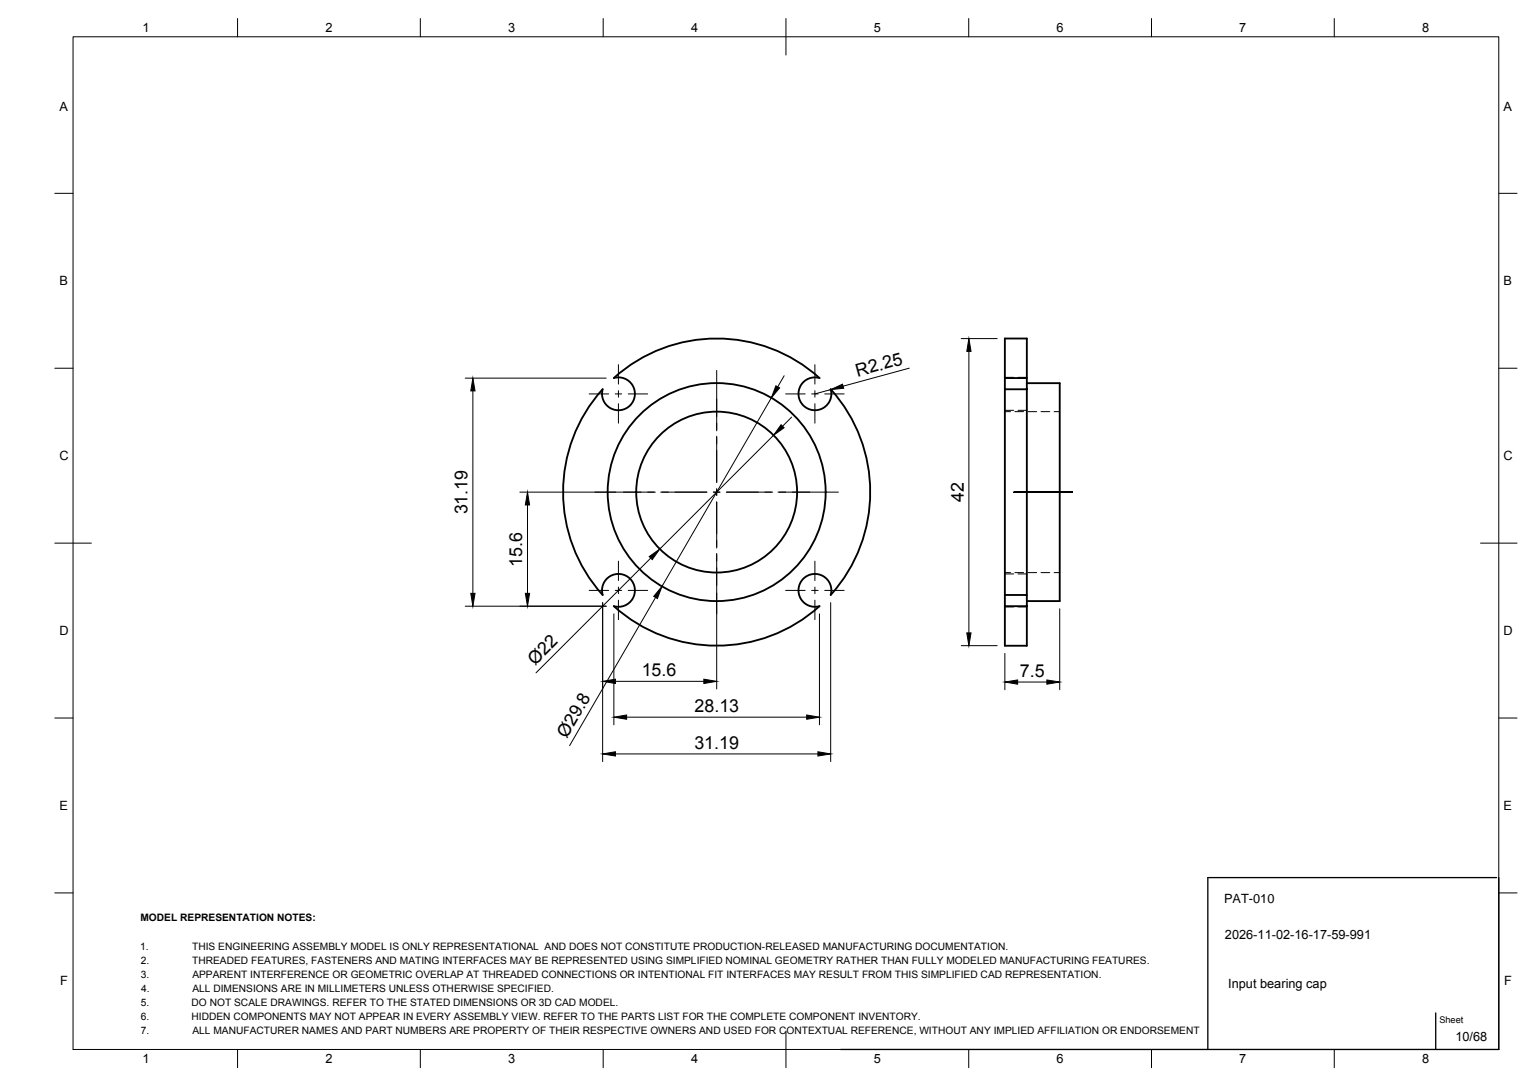
ISO-10303-21;
HEADER;
/* Generated by software containing ST-Developer
 * from STEP Tools, Inc. (www.steptools.com) 
 */

FILE_DESCRIPTION(
/* description */ ('Belt conveyor head drive unit'),
/* implementation_level */ '2;1');

FILE_NAME(
/* name */ 'Input bearing cap.step',
/* time_stamp */ '2026-10-28T03:26:19-07:00',
/* author */ (''),
/* organization */ (''),
/* preprocessor_version */ 'ST-DEVELOPER v20.2',
/* originating_system */ 'Autodesk Translation Framework v15.17.0.0',
/* authorisation */ '');

FILE_SCHEMA (('AUTOMOTIVE_DESIGN { 1 0 10303 214 3 1 1 }'));
ENDSEC;

DATA;
#10=MECHANICAL_DESIGN_GEOMETRIC_PRESENTATION_REPRESENTATION('',(#852),#27069);
#714=SHAPE_REPRESENTATION_RELATIONSHIP('SRR','None',#27358,#783);
#783=ADVANCED_BREP_SHAPE_REPRESENTATION('',(#937),#27000);
#852=STYLED_ITEM('',(#27797),#937);
#937=MANIFOLD_SOLID_BREP('Body1',#13717);
#1052=FACE_BOUND('',#2563,.T.);
#1053=FACE_BOUND('',#2570,.T.);
#1054=FACE_BOUND('',#2573,.T.);
#1329=PLANE('',#14737);
#1330=PLANE('',#14754);
#1331=PLANE('',#14757);
#1718=FACE_OUTER_BOUND('',#2558,.T.);
#1719=FACE_OUTER_BOUND('',#2559,.T.);
#1720=FACE_OUTER_BOUND('',#2560,.T.);
#1721=FACE_OUTER_BOUND('',#2561,.T.);
#1722=FACE_OUTER_BOUND('',#2562,.T.);
#1723=FACE_OUTER_BOUND('',#2564,.T.);
#1724=FACE_OUTER_BOUND('',#2565,.T.);
#1725=FACE_OUTER_BOUND('',#2566,.T.);
#1726=FACE_OUTER_BOUND('',#2567,.T.);
#1727=FACE_OUTER_BOUND('',#2568,.T.);
#1728=FACE_OUTER_BOUND('',#2569,.T.);
#1729=FACE_OUTER_BOUND('',#2571,.T.);
#1730=FACE_OUTER_BOUND('',#2572,.T.);
#2558=EDGE_LOOP('',(#9336,#9337,#9338,#9339));
#2559=EDGE_LOOP('',(#9340,#9341,#9342,#9343));
#2560=EDGE_LOOP('',(#9344,#9345,#9346,#9347));
#2561=EDGE_LOOP('',(#9348,#9349,#9350,#9351));
#2562=EDGE_LOOP('',(#9352,#9353,#9354,#9355,#9356,#9357,#9358,#9359));
#2563=EDGE_LOOP('',(#9360));
#2564=EDGE_LOOP('',(#9361,#9362,#9363,#9364));
#2565=EDGE_LOOP('',(#9365,#9366,#9367,#9368));
#2566=EDGE_LOOP('',(#9369,#9370,#9371,#9372));
#2567=EDGE_LOOP('',(#9373,#9374,#9375,#9376));
#2568=EDGE_LOOP('',(#9377,#9378,#9379,#9380));
#2569=EDGE_LOOP('',(#9381));
#2570=EDGE_LOOP('',(#9382));
#2571=EDGE_LOOP('',(#9383,#9384,#9385,#9386));
#2572=EDGE_LOOP('',(#9387,#9388,#9389,#9390,#9391,#9392,#9393,#9394));
#2573=EDGE_LOOP('',(#9395));
#3617=LINE('',#21381,#4409);
#3618=LINE('',#21385,#4410);
#3619=LINE('',#21390,#4411);
#3620=LINE('',#21394,#4412);
#3621=LINE('',#21399,#4413);
#3622=LINE('',#21403,#4414);
#3623=LINE('',#21408,#4415);
#3624=LINE('',#21412,#4416);
#3625=LINE('',#21433,#4417);
#3626=LINE('',#21439,#4418);
#4409=VECTOR('',#16881,1.);
#4410=VECTOR('',#16884,1.);
#4411=VECTOR('',#16889,1.);
#4412=VECTOR('',#16892,1.);
#4413=VECTOR('',#16897,1.);
#4414=VECTOR('',#16900,1.);
#4415=VECTOR('',#16905,1.);
#4416=VECTOR('',#16908,1.);
#4417=VECTOR('',#16943,1.49);
#4418=VECTOR('',#16952,1.1);
#5152=CIRCLE('',#14726,0.225);
#5153=CIRCLE('',#14727,0.225);
#5154=CIRCLE('',#14729,0.225);
#5155=CIRCLE('',#14730,0.225);
#5156=CIRCLE('',#14732,0.225);
#5157=CIRCLE('',#14733,0.225);
#5158=CIRCLE('',#14735,0.225);
#5159=CIRCLE('',#14736,0.225);
#5160=CIRCLE('',#14738,2.1);
#5161=CIRCLE('',#14739,2.1);
#5162=CIRCLE('',#14740,2.1);
#5163=CIRCLE('',#14741,2.1);
#5164=CIRCLE('',#14742,1.1);
#5165=CIRCLE('',#14744,2.1);
#5166=CIRCLE('',#14746,2.1);
#5167=CIRCLE('',#14748,2.1);
#5168=CIRCLE('',#14750,2.1);
#5169=CIRCLE('',#14752,1.49);
#5170=CIRCLE('',#14753,1.49);
#5171=CIRCLE('',#14755,1.1);
#6079=VERTEX_POINT('',#21379);
#6080=VERTEX_POINT('',#21380);
#6081=VERTEX_POINT('',#21382);
#6082=VERTEX_POINT('',#21384);
#6083=VERTEX_POINT('',#21388);
#6084=VERTEX_POINT('',#21389);
#6085=VERTEX_POINT('',#21391);
#6086=VERTEX_POINT('',#21393);
#6087=VERTEX_POINT('',#21397);
#6088=VERTEX_POINT('',#21398);
#6089=VERTEX_POINT('',#21400);
#6090=VERTEX_POINT('',#21402);
#6091=VERTEX_POINT('',#21406);
#6092=VERTEX_POINT('',#21407);
#6093=VERTEX_POINT('',#21409);
#6094=VERTEX_POINT('',#21411);
#6095=VERTEX_POINT('',#21419);
#6096=VERTEX_POINT('',#21430);
#6097=VERTEX_POINT('',#21432);
#6098=VERTEX_POINT('',#21436);
#7360=EDGE_CURVE('',#6079,#6080,#3617,.T.);
#7361=EDGE_CURVE('',#6081,#6079,#5152,.T.);
#7362=EDGE_CURVE('',#6082,#6081,#3618,.T.);
#7363=EDGE_CURVE('',#6080,#6082,#5153,.T.);
#7364=EDGE_CURVE('',#6083,#6084,#3619,.T.);
#7365=EDGE_CURVE('',#6085,#6083,#5154,.T.);
#7366=EDGE_CURVE('',#6086,#6085,#3620,.T.);
#7367=EDGE_CURVE('',#6084,#6086,#5155,.T.);
#7368=EDGE_CURVE('',#6087,#6088,#3621,.T.);
#7369=EDGE_CURVE('',#6089,#6087,#5156,.T.);
#7370=EDGE_CURVE('',#6090,#6089,#3622,.T.);
#7371=EDGE_CURVE('',#6088,#6090,#5157,.T.);
#7372=EDGE_CURVE('',#6091,#6092,#3623,.T.);
#7373=EDGE_CURVE('',#6093,#6091,#5158,.T.);
#7374=EDGE_CURVE('',#6094,#6093,#3624,.T.);
#7375=EDGE_CURVE('',#6092,#6094,#5159,.T.);
#7376=EDGE_CURVE('',#6093,#6079,#5160,.T.);
#7377=EDGE_CURVE('',#6089,#6091,#5161,.T.);
#7378=EDGE_CURVE('',#6085,#6087,#5162,.T.);
#7379=EDGE_CURVE('',#6081,#6083,#5163,.T.);
#7380=EDGE_CURVE('',#6095,#6095,#5164,.T.);
#7381=EDGE_CURVE('',#6090,#6092,#5165,.T.);
#7382=EDGE_CURVE('',#6086,#6088,#5166,.T.);
#7383=EDGE_CURVE('',#6094,#6080,#5167,.T.);
#7384=EDGE_CURVE('',#6082,#6084,#5168,.T.);
#7385=EDGE_CURVE('',#6096,#6096,#5169,.T.);
#7386=EDGE_CURVE('',#6096,#6097,#3625,.T.);
#7387=EDGE_CURVE('',#6097,#6097,#5170,.T.);
#7388=EDGE_CURVE('',#6098,#6098,#5171,.T.);
#7389=EDGE_CURVE('',#6098,#6095,#3626,.T.);
#9336=ORIENTED_EDGE('',*,*,#7360,.F.);
#9337=ORIENTED_EDGE('',*,*,#7361,.F.);
#9338=ORIENTED_EDGE('',*,*,#7362,.F.);
#9339=ORIENTED_EDGE('',*,*,#7363,.F.);
#9340=ORIENTED_EDGE('',*,*,#7364,.F.);
#9341=ORIENTED_EDGE('',*,*,#7365,.F.);
#9342=ORIENTED_EDGE('',*,*,#7366,.F.);
#9343=ORIENTED_EDGE('',*,*,#7367,.F.);
#9344=ORIENTED_EDGE('',*,*,#7368,.F.);
#9345=ORIENTED_EDGE('',*,*,#7369,.F.);
#9346=ORIENTED_EDGE('',*,*,#7370,.F.);
#9347=ORIENTED_EDGE('',*,*,#7371,.F.);
#9348=ORIENTED_EDGE('',*,*,#7372,.F.);
#9349=ORIENTED_EDGE('',*,*,#7373,.F.);
#9350=ORIENTED_EDGE('',*,*,#7374,.F.);
#9351=ORIENTED_EDGE('',*,*,#7375,.F.);
#9352=ORIENTED_EDGE('',*,*,#7361,.T.);
#9353=ORIENTED_EDGE('',*,*,#7376,.F.);
#9354=ORIENTED_EDGE('',*,*,#7373,.T.);
#9355=ORIENTED_EDGE('',*,*,#7377,.F.);
#9356=ORIENTED_EDGE('',*,*,#7369,.T.);
#9357=ORIENTED_EDGE('',*,*,#7378,.F.);
#9358=ORIENTED_EDGE('',*,*,#7365,.T.);
#9359=ORIENTED_EDGE('',*,*,#7379,.F.);
#9360=ORIENTED_EDGE('',*,*,#7380,.F.);
#9361=ORIENTED_EDGE('',*,*,#7370,.T.);
#9362=ORIENTED_EDGE('',*,*,#7377,.T.);
#9363=ORIENTED_EDGE('',*,*,#7372,.T.);
#9364=ORIENTED_EDGE('',*,*,#7381,.F.);
#9365=ORIENTED_EDGE('',*,*,#7366,.T.);
#9366=ORIENTED_EDGE('',*,*,#7378,.T.);
#9367=ORIENTED_EDGE('',*,*,#7368,.T.);
#9368=ORIENTED_EDGE('',*,*,#7382,.F.);
#9369=ORIENTED_EDGE('',*,*,#7360,.T.);
#9370=ORIENTED_EDGE('',*,*,#7383,.F.);
#9371=ORIENTED_EDGE('',*,*,#7374,.T.);
#9372=ORIENTED_EDGE('',*,*,#7376,.T.);
#9373=ORIENTED_EDGE('',*,*,#7362,.T.);
#9374=ORIENTED_EDGE('',*,*,#7379,.T.);
#9375=ORIENTED_EDGE('',*,*,#7364,.T.);
#9376=ORIENTED_EDGE('',*,*,#7384,.F.);
#9377=ORIENTED_EDGE('',*,*,#7385,.F.);
#9378=ORIENTED_EDGE('',*,*,#7386,.T.);
#9379=ORIENTED_EDGE('',*,*,#7387,.F.);
#9380=ORIENTED_EDGE('',*,*,#7386,.F.);
#9381=ORIENTED_EDGE('',*,*,#7385,.T.);
#9382=ORIENTED_EDGE('',*,*,#7388,.T.);
#9383=ORIENTED_EDGE('',*,*,#7388,.F.);
#9384=ORIENTED_EDGE('',*,*,#7389,.T.);
#9385=ORIENTED_EDGE('',*,*,#7380,.T.);
#9386=ORIENTED_EDGE('',*,*,#7389,.F.);
#9387=ORIENTED_EDGE('',*,*,#7363,.T.);
#9388=ORIENTED_EDGE('',*,*,#7384,.T.);
#9389=ORIENTED_EDGE('',*,*,#7367,.T.);
#9390=ORIENTED_EDGE('',*,*,#7382,.T.);
#9391=ORIENTED_EDGE('',*,*,#7371,.T.);
#9392=ORIENTED_EDGE('',*,*,#7381,.T.);
#9393=ORIENTED_EDGE('',*,*,#7375,.T.);
#9394=ORIENTED_EDGE('',*,*,#7383,.T.);
#9395=ORIENTED_EDGE('',*,*,#7387,.T.);
#12565=CYLINDRICAL_SURFACE('',#14725,0.225);
#12566=CYLINDRICAL_SURFACE('',#14728,0.225);
#12567=CYLINDRICAL_SURFACE('',#14731,0.225);
#12568=CYLINDRICAL_SURFACE('',#14734,0.225);
#12569=CYLINDRICAL_SURFACE('',#14743,2.1);
#12570=CYLINDRICAL_SURFACE('',#14745,2.1);
#12571=CYLINDRICAL_SURFACE('',#14747,2.1);
#12572=CYLINDRICAL_SURFACE('',#14749,2.1);
#12573=CYLINDRICAL_SURFACE('',#14751,1.49);
#12574=CYLINDRICAL_SURFACE('',#14756,1.1);
#12997=ADVANCED_FACE('',(#1718),#12565,.F.);
#12998=ADVANCED_FACE('',(#1719),#12566,.F.);
#12999=ADVANCED_FACE('',(#1720),#12567,.F.);
#13000=ADVANCED_FACE('',(#1721),#12568,.F.);
#13001=ADVANCED_FACE('',(#1722,#1052),#1329,.F.);
#13002=ADVANCED_FACE('',(#1723),#12569,.T.);
#13003=ADVANCED_FACE('',(#1724),#12570,.T.);
#13004=ADVANCED_FACE('',(#1725),#12571,.T.);
#13005=ADVANCED_FACE('',(#1726),#12572,.T.);
#13006=ADVANCED_FACE('',(#1727),#12573,.T.);
#13007=ADVANCED_FACE('',(#1728,#1053),#1330,.T.);
#13008=ADVANCED_FACE('',(#1729),#12574,.F.);
#13009=ADVANCED_FACE('',(#1730,#1054),#1331,.T.);
#13717=CLOSED_SHELL('',(#12997,#12998,#12999,#13000,#13001,#13002,#13003,
#13004,#13005,#13006,#13007,#13008,#13009));
#14724=AXIS2_PLACEMENT_3D('',#21377,#16877,#16878);
#14725=AXIS2_PLACEMENT_3D('',#21378,#16879,#16880);
#14726=AXIS2_PLACEMENT_3D('',#21383,#16882,#16883);
#14727=AXIS2_PLACEMENT_3D('',#21386,#16885,#16886);
#14728=AXIS2_PLACEMENT_3D('',#21387,#16887,#16888);
#14729=AXIS2_PLACEMENT_3D('',#21392,#16890,#16891);
#14730=AXIS2_PLACEMENT_3D('',#21395,#16893,#16894);
#14731=AXIS2_PLACEMENT_3D('',#21396,#16895,#16896);
#14732=AXIS2_PLACEMENT_3D('',#21401,#16898,#16899);
#14733=AXIS2_PLACEMENT_3D('',#21404,#16901,#16902);
#14734=AXIS2_PLACEMENT_3D('',#21405,#16903,#16904);
#14735=AXIS2_PLACEMENT_3D('',#21410,#16906,#16907);
#14736=AXIS2_PLACEMENT_3D('',#21413,#16909,#16910);
#14737=AXIS2_PLACEMENT_3D('',#21414,#16911,#16912);
#14738=AXIS2_PLACEMENT_3D('',#21415,#16913,#16914);
#14739=AXIS2_PLACEMENT_3D('',#21416,#16915,#16916);
#14740=AXIS2_PLACEMENT_3D('',#21417,#16917,#16918);
#14741=AXIS2_PLACEMENT_3D('',#21418,#16919,#16920);
#14742=AXIS2_PLACEMENT_3D('',#21420,#16921,#16922);
#14743=AXIS2_PLACEMENT_3D('',#21421,#16923,#16924);
#14744=AXIS2_PLACEMENT_3D('',#21422,#16925,#16926);
#14745=AXIS2_PLACEMENT_3D('',#21423,#16927,#16928);
#14746=AXIS2_PLACEMENT_3D('',#21424,#16929,#16930);
#14747=AXIS2_PLACEMENT_3D('',#21425,#16931,#16932);
#14748=AXIS2_PLACEMENT_3D('',#21426,#16933,#16934);
#14749=AXIS2_PLACEMENT_3D('',#21427,#16935,#16936);
#14750=AXIS2_PLACEMENT_3D('',#21428,#16937,#16938);
#14751=AXIS2_PLACEMENT_3D('',#21429,#16939,#16940);
#14752=AXIS2_PLACEMENT_3D('',#21431,#16941,#16942);
#14753=AXIS2_PLACEMENT_3D('',#21434,#16944,#16945);
#14754=AXIS2_PLACEMENT_3D('',#21435,#16946,#16947);
#14755=AXIS2_PLACEMENT_3D('',#21437,#16948,#16949);
#14756=AXIS2_PLACEMENT_3D('',#21438,#16950,#16951);
#14757=AXIS2_PLACEMENT_3D('',#21440,#16953,#16954);
#16877=DIRECTION('axis',(0.,0.,1.));
#16878=DIRECTION('refdir',(1.,0.,0.));
#16879=DIRECTION('center_axis',(0.,1.,0.));
#16880=DIRECTION('ref_axis',(0.707106781186546,0.,0.707106781186549));
#16881=DIRECTION('',(0.,1.,0.));
#16882=DIRECTION('center_axis',(0.,1.,0.));
#16883=DIRECTION('ref_axis',(1.,0.,0.));
#16884=DIRECTION('',(0.,-1.,0.));
#16885=DIRECTION('center_axis',(0.,-1.,0.));
#16886=DIRECTION('ref_axis',(1.,0.,0.));
#16887=DIRECTION('center_axis',(0.,1.,0.));
#16888=DIRECTION('ref_axis',(0.707106781186547,0.,-0.707106781186548));
#16889=DIRECTION('',(0.,1.,0.));
#16890=DIRECTION('center_axis',(0.,1.,0.));
#16891=DIRECTION('ref_axis',(1.,0.,0.));
#16892=DIRECTION('',(0.,-1.,0.));
#16893=DIRECTION('center_axis',(0.,-1.,0.));
#16894=DIRECTION('ref_axis',(1.,0.,0.));
#16895=DIRECTION('center_axis',(0.,1.,0.));
#16896=DIRECTION('ref_axis',(-0.707106781186552,0.,-0.707106781186543));
#16897=DIRECTION('',(0.,1.,0.));
#16898=DIRECTION('center_axis',(0.,1.,0.));
#16899=DIRECTION('ref_axis',(1.,0.,0.));
#16900=DIRECTION('',(0.,-1.,0.));
#16901=DIRECTION('center_axis',(0.,-1.,0.));
#16902=DIRECTION('ref_axis',(1.,0.,0.));
#16903=DIRECTION('center_axis',(0.,1.,0.));
#16904=DIRECTION('ref_axis',(-0.707106781186546,0.,0.707106781186549));
#16905=DIRECTION('',(0.,1.,0.));
#16906=DIRECTION('center_axis',(0.,1.,0.));
#16907=DIRECTION('ref_axis',(1.,0.,0.));
#16908=DIRECTION('',(0.,-1.,0.));
#16909=DIRECTION('center_axis',(0.,-1.,0.));
#16910=DIRECTION('ref_axis',(1.,0.,0.));
#16911=DIRECTION('center_axis',(0.,1.,0.));
#16912=DIRECTION('ref_axis',(1.,0.,0.));
#16913=DIRECTION('center_axis',(0.,1.,0.));
#16914=DIRECTION('ref_axis',(1.,0.,0.));
#16915=DIRECTION('center_axis',(0.,1.,0.));
#16916=DIRECTION('ref_axis',(1.,0.,0.));
#16917=DIRECTION('center_axis',(0.,1.,0.));
#16918=DIRECTION('ref_axis',(1.,0.,0.));
#16919=DIRECTION('center_axis',(0.,1.,0.));
#16920=DIRECTION('ref_axis',(1.,0.,0.));
#16921=DIRECTION('center_axis',(0.,-1.,0.));
#16922=DIRECTION('ref_axis',(1.,0.,0.));
#16923=DIRECTION('center_axis',(0.,1.,0.));
#16924=DIRECTION('ref_axis',(1.,0.,0.));
#16925=DIRECTION('center_axis',(0.,1.,0.));
#16926=DIRECTION('ref_axis',(1.,0.,0.));
#16927=DIRECTION('center_axis',(0.,1.,0.));
#16928=DIRECTION('ref_axis',(1.,0.,0.));
#16929=DIRECTION('center_axis',(0.,1.,0.));
#16930=DIRECTION('ref_axis',(1.,0.,0.));
#16931=DIRECTION('center_axis',(0.,1.,0.));
#16932=DIRECTION('ref_axis',(1.,0.,0.));
#16933=DIRECTION('center_axis',(0.,1.,0.));
#16934=DIRECTION('ref_axis',(1.,0.,0.));
#16935=DIRECTION('center_axis',(0.,1.,0.));
#16936=DIRECTION('ref_axis',(-1.,0.,-1.22464679914735E-16));
#16937=DIRECTION('center_axis',(0.,1.,0.));
#16938=DIRECTION('ref_axis',(1.,0.,0.));
#16939=DIRECTION('center_axis',(0.,1.,0.));
#16940=DIRECTION('ref_axis',(1.,0.,0.));
#16941=DIRECTION('center_axis',(0.,1.,0.));
#16942=DIRECTION('ref_axis',(1.,0.,0.));
#16943=DIRECTION('',(0.,-1.,0.));
#16944=DIRECTION('center_axis',(0.,-1.,0.));
#16945=DIRECTION('ref_axis',(1.,0.,0.));
#16946=DIRECTION('center_axis',(0.,1.,0.));
#16947=DIRECTION('ref_axis',(1.,0.,0.));
#16948=DIRECTION('center_axis',(0.,-1.,0.));
#16949=DIRECTION('ref_axis',(1.,0.,0.));
#16950=DIRECTION('center_axis',(0.,1.,0.));
#16951=DIRECTION('ref_axis',(1.,0.,0.));
#16952=DIRECTION('',(0.,-1.,0.));
#16953=DIRECTION('center_axis',(0.,1.,0.));
#16954=DIRECTION('ref_axis',(1.,0.,0.));
#21377=CARTESIAN_POINT('',(0.,0.,0.));
#21378=CARTESIAN_POINT('Origin',(-1.34350288425444,-2.2,5.65649711574556));
#21379=CARTESIAN_POINT('',(-1.40634555589641,-2.1,5.4404512904656));
#21380=CARTESIAN_POINT('',(-1.40634555589641,-1.8,5.4404512904656));
#21381=CARTESIAN_POINT('',(-1.40634555589641,-2.2,5.4404512904656));
#21382=CARTESIAN_POINT('',(-1.5595487095344,-2.1,5.59365444410359));
#21383=CARTESIAN_POINT('Origin',(-1.34350288425444,-2.1,5.65649711574556));
#21384=CARTESIAN_POINT('',(-1.5595487095344,-1.8,5.59365444410359));
#21385=CARTESIAN_POINT('',(-1.5595487095344,-2.2,5.59365444410359));
#21386=CARTESIAN_POINT('Origin',(-1.34350288425444,-1.8,5.65649711574556));
#21387=CARTESIAN_POINT('Origin',(-1.34350288425444,-2.2,8.34350288425444));
#21388=CARTESIAN_POINT('',(-1.5595487095344,-2.1,8.40634555589641));
#21389=CARTESIAN_POINT('',(-1.5595487095344,-1.8,8.40634555589641));
#21390=CARTESIAN_POINT('',(-1.5595487095344,-2.2,8.40634555589641));
#21391=CARTESIAN_POINT('',(-1.40634555589641,-2.1,8.5595487095344));
#21392=CARTESIAN_POINT('Origin',(-1.34350288425444,-2.1,8.34350288425444));
#21393=CARTESIAN_POINT('',(-1.40634555589641,-1.8,8.5595487095344));
#21394=CARTESIAN_POINT('',(-1.40634555589641,-2.2,8.5595487095344));
#21395=CARTESIAN_POINT('Origin',(-1.34350288425444,-1.8,8.34350288425444));
#21396=CARTESIAN_POINT('Origin',(1.34350288425444,-2.2,8.34350288425444));
#21397=CARTESIAN_POINT('',(1.40634555589641,-2.1,8.5595487095344));
#21398=CARTESIAN_POINT('',(1.40634555589641,-1.8,8.5595487095344));
#21399=CARTESIAN_POINT('',(1.40634555589641,-2.2,8.5595487095344));
#21400=CARTESIAN_POINT('',(1.5595487095344,-2.1,8.40634555589641));
#21401=CARTESIAN_POINT('Origin',(1.34350288425444,-2.1,8.34350288425444));
#21402=CARTESIAN_POINT('',(1.5595487095344,-1.8,8.40634555589641));
#21403=CARTESIAN_POINT('',(1.5595487095344,-2.2,8.40634555589641));
#21404=CARTESIAN_POINT('Origin',(1.34350288425444,-1.8,8.34350288425444));
#21405=CARTESIAN_POINT('Origin',(1.34350288425444,-2.2,5.65649711574556));
#21406=CARTESIAN_POINT('',(1.5595487095344,-2.1,5.59365444410359));
#21407=CARTESIAN_POINT('',(1.5595487095344,-1.8,5.59365444410359));
#21408=CARTESIAN_POINT('',(1.5595487095344,-2.2,5.59365444410359));
#21409=CARTESIAN_POINT('',(1.40634555589641,-2.1,5.4404512904656));
#21410=CARTESIAN_POINT('Origin',(1.34350288425444,-2.1,5.65649711574556));
#21411=CARTESIAN_POINT('',(1.40634555589641,-1.8,5.4404512904656));
#21412=CARTESIAN_POINT('',(1.40634555589641,-2.2,5.4404512904656));
#21413=CARTESIAN_POINT('Origin',(1.34350288425444,-1.8,5.65649711574556));
#21414=CARTESIAN_POINT('Origin',(0.,-2.1,7.));
#21415=CARTESIAN_POINT('Origin',(0.,-2.1,7.));
#21416=CARTESIAN_POINT('Origin',(0.,-2.1,7.));
#21417=CARTESIAN_POINT('Origin',(0.,-2.1,7.));
#21418=CARTESIAN_POINT('Origin',(0.,-2.1,7.));
#21419=CARTESIAN_POINT('',(-1.1,-2.1,7.));
#21420=CARTESIAN_POINT('Origin',(0.,-2.1,7.));
#21421=CARTESIAN_POINT('Origin',(0.,-2.1,7.));
#21422=CARTESIAN_POINT('Origin',(0.,-1.8,7.));
#21423=CARTESIAN_POINT('Origin',(0.,-2.1,7.));
#21424=CARTESIAN_POINT('Origin',(0.,-1.8,7.));
#21425=CARTESIAN_POINT('Origin',(0.,-2.1,7.));
#21426=CARTESIAN_POINT('Origin',(0.,-1.8,7.));
#21427=CARTESIAN_POINT('Origin',(0.,-2.1,7.));
#21428=CARTESIAN_POINT('Origin',(0.,-1.8,7.));
#21429=CARTESIAN_POINT('Origin',(0.,-1.8,7.));
#21430=CARTESIAN_POINT('',(-1.49,-1.35,7.));
#21431=CARTESIAN_POINT('Origin',(0.,-1.35,7.));
#21432=CARTESIAN_POINT('',(-1.49,-1.8,7.));
#21433=CARTESIAN_POINT('',(-1.49,-1.8,7.));
#21434=CARTESIAN_POINT('Origin',(0.,-1.8,7.));
#21435=CARTESIAN_POINT('Origin',(0.,-1.35,7.));
#21436=CARTESIAN_POINT('',(-1.1,-1.35,7.));
#21437=CARTESIAN_POINT('Origin',(0.,-1.35,7.));
#21438=CARTESIAN_POINT('Origin',(0.,-2.1,7.));
#21439=CARTESIAN_POINT('',(-1.1,-2.1,7.));
#21440=CARTESIAN_POINT('Origin',(0.,-1.8,7.));
#26923=UNCERTAINTY_MEASURE_WITH_UNIT(LENGTH_MEASURE(0.001),#27070,
'DISTANCE_ACCURACY_VALUE',
'Maximum model space distance between geometric entities at asserted c
onnectivities');
#26992=UNCERTAINTY_MEASURE_WITH_UNIT(LENGTH_MEASURE(0.001),#27070,
'DISTANCE_ACCURACY_VALUE',
'Maximum model space distance between geometric entities at asserted c
onnectivities');
#27000=(
GEOMETRIC_REPRESENTATION_CONTEXT(3)
GLOBAL_UNCERTAINTY_ASSIGNED_CONTEXT((#26923))
GLOBAL_UNIT_ASSIGNED_CONTEXT((#27070,#27072,#27073))
REPRESENTATION_CONTEXT('','3D')
);
#27069=(
GEOMETRIC_REPRESENTATION_CONTEXT(3)
GLOBAL_UNCERTAINTY_ASSIGNED_CONTEXT((#26992))
GLOBAL_UNIT_ASSIGNED_CONTEXT((#27070,#27072,#27073))
REPRESENTATION_CONTEXT('','3D')
);
#27070=(
LENGTH_UNIT()
NAMED_UNIT(*)
SI_UNIT(.CENTI.,.METRE.)
);
#27072=(
NAMED_UNIT(*)
PLANE_ANGLE_UNIT()
SI_UNIT($,.RADIAN.)
);
#27073=(
NAMED_UNIT(*)
SI_UNIT($,.STERADIAN.)
SOLID_ANGLE_UNIT()
);
#27081=SHAPE_DEFINITION_REPRESENTATION(#27157,#27358);
#27157=PRODUCT_DEFINITION_SHAPE('',$,#27435);
#27358=SHAPE_REPRESENTATION('',(#14724),#27000);
#27427=PRODUCT_DEFINITION_CONTEXT('part definition',#27657,'design');
#27435=PRODUCT_DEFINITION('Input bearing cap','Input bearing cap',#27511,
#27427);
#27511=PRODUCT_DEFINITION_FORMATION('',$,#27666);
#27657=APPLICATION_CONTEXT(
'Core Data for Automotive Mechanical Design Process');
#27658=PRODUCT_CONTEXT('part definition',#27657,'mechanical');
#27666=PRODUCT('Input bearing cap','Input bearing cap',
'Input bearing cap',(#27658));
#27791=COLOUR_RGB('Grey',0.48,0.52,0.57);
#27792=FILL_AREA_STYLE_COLOUR('',#27791);
#27793=FILL_AREA_STYLE('',(#27792));
#27794=SURFACE_STYLE_FILL_AREA(#27793);
#27795=SURFACE_SIDE_STYLE('',(#27794));
#27796=SURFACE_STYLE_USAGE(.BOTH.,#27795);
#27797=PRESENTATION_STYLE_ASSIGNMENT((#27796));
ENDSEC;
END-ISO-10303-21;
